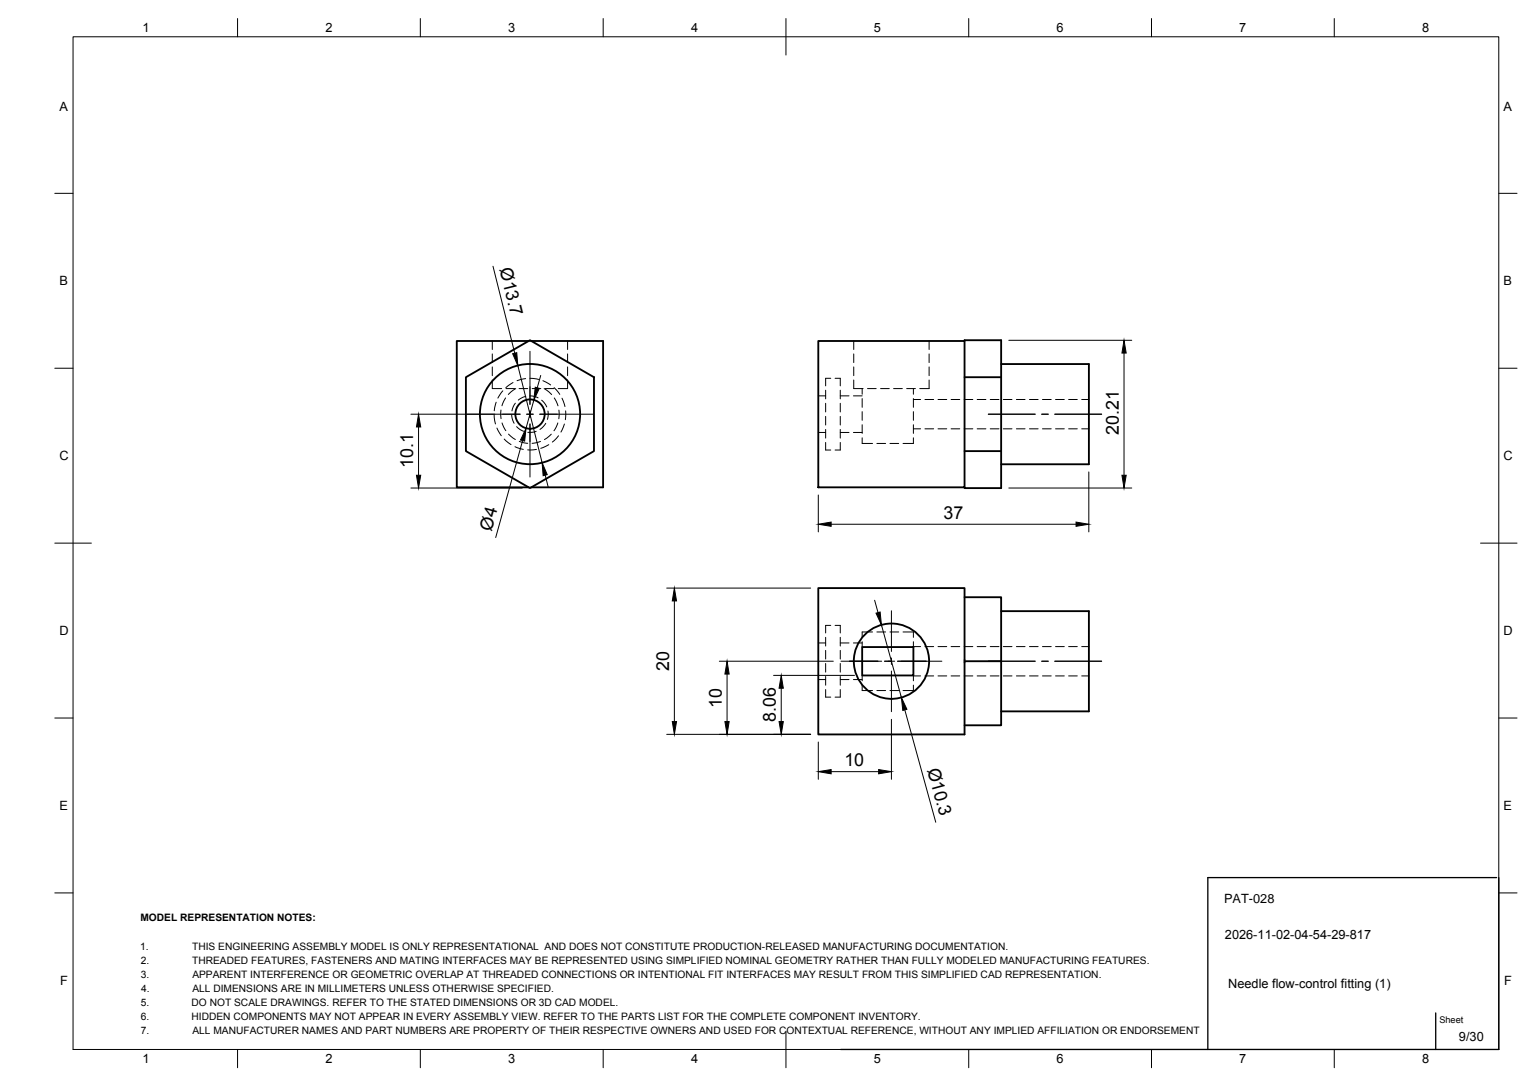
ISO-10303-21;
HEADER;
/* Generated by software containing ST-Developer
 * from STEP Tools, Inc. (www.steptools.com) 
 */

FILE_DESCRIPTION(
/* description */ ('Cylinder foot and clevis mount kit'),
/* implementation_level */ '2;1');

FILE_NAME(
/* name */ 'Needle flow-control fitting (1).step',
/* time_stamp */ '2026-10-27T20:10:43-07:00',
/* author */ (''),
/* organization */ (''),
/* preprocessor_version */ 'ST-DEVELOPER v20.2',
/* originating_system */ 'Autodesk Translation Framework v15.17.0.0',
/* authorisation */ '');

FILE_SCHEMA (('AUTOMOTIVE_DESIGN { 1 0 10303 214 3 1 1 }'));
ENDSEC;

DATA;
#10=MECHANICAL_DESIGN_GEOMETRIC_PRESENTATION_REPRESENTATION('',(#342),#9102);
#286=SHAPE_REPRESENTATION_RELATIONSHIP('SRR','None',#9233,#314);
#314=ADVANCED_BREP_SHAPE_REPRESENTATION('',(#370),#9076);
#342=STYLED_ITEM('',(#9453),#370);
#370=MANIFOLD_SOLID_BREP('Body1',#4928);
#430=FACE_BOUND('',#1139,.T.);
#431=FACE_BOUND('',#1141,.T.);
#432=FACE_BOUND('',#1145,.T.);
#433=FACE_BOUND('',#1147,.T.);
#434=FACE_BOUND('',#1151,.T.);
#435=FACE_BOUND('',#1155,.T.);
#436=FACE_BOUND('',#1159,.T.);
#437=FACE_BOUND('',#1163,.T.);
#438=FACE_BOUND('',#1174,.T.);
#567=PLANE('',#5462);
#568=PLANE('',#5463);
#569=PLANE('',#5471);
#570=PLANE('',#5473);
#571=PLANE('',#5478);
#572=PLANE('',#5480);
#573=PLANE('',#5481);
#574=PLANE('',#5482);
#575=PLANE('',#5483);
#576=PLANE('',#5484);
#577=PLANE('',#5485);
#578=PLANE('',#5486);
#579=PLANE('',#5487);
#580=PLANE('',#5488);
#581=PLANE('',#5490);
#582=PLANE('',#5491);
#583=PLANE('',#5492);
#584=PLANE('',#5493);
#585=PLANE('',#5494);
#586=PLANE('',#5495);
#587=PLANE('',#5496);
#588=PLANE('',#5501);
#793=FACE_OUTER_BOUND('',#1137,.T.);
#794=FACE_OUTER_BOUND('',#1138,.T.);
#795=FACE_OUTER_BOUND('',#1140,.T.);
#796=FACE_OUTER_BOUND('',#1142,.T.);
#797=FACE_OUTER_BOUND('',#1143,.T.);
#798=FACE_OUTER_BOUND('',#1144,.T.);
#799=FACE_OUTER_BOUND('',#1146,.T.);
#800=FACE_OUTER_BOUND('',#1148,.T.);
#801=FACE_OUTER_BOUND('',#1149,.T.);
#802=FACE_OUTER_BOUND('',#1150,.T.);
#803=FACE_OUTER_BOUND('',#1152,.T.);
#804=FACE_OUTER_BOUND('',#1153,.T.);
#805=FACE_OUTER_BOUND('',#1154,.T.);
#806=FACE_OUTER_BOUND('',#1156,.T.);
#807=FACE_OUTER_BOUND('',#1157,.T.);
#808=FACE_OUTER_BOUND('',#1158,.T.);
#809=FACE_OUTER_BOUND('',#1160,.T.);
#810=FACE_OUTER_BOUND('',#1161,.T.);
#811=FACE_OUTER_BOUND('',#1162,.T.);
#812=FACE_OUTER_BOUND('',#1164,.T.);
#813=FACE_OUTER_BOUND('',#1165,.T.);
#814=FACE_OUTER_BOUND('',#1166,.T.);
#815=FACE_OUTER_BOUND('',#1167,.T.);
#816=FACE_OUTER_BOUND('',#1168,.T.);
#817=FACE_OUTER_BOUND('',#1169,.T.);
#818=FACE_OUTER_BOUND('',#1170,.T.);
#819=FACE_OUTER_BOUND('',#1171,.T.);
#820=FACE_OUTER_BOUND('',#1172,.T.);
#821=FACE_OUTER_BOUND('',#1173,.T.);
#1137=EDGE_LOOP('',(#3719,#3720,#3721,#3722));
#1138=EDGE_LOOP('',(#3723));
#1139=EDGE_LOOP('',(#3724,#3725,#3726,#3727));
#1140=EDGE_LOOP('',(#3728,#3729));
#1141=EDGE_LOOP('',(#3730));
#1142=EDGE_LOOP('',(#3731,#3732,#3733,#3734));
#1143=EDGE_LOOP('',(#3735,#3736,#3737,#3738));
#1144=EDGE_LOOP('',(#3739));
#1145=EDGE_LOOP('',(#3740));
#1146=EDGE_LOOP('',(#3741));
#1147=EDGE_LOOP('',(#3742));
#1148=EDGE_LOOP('',(#3743,#3744,#3745,#3746));
#1149=EDGE_LOOP('',(#3747,#3748,#3749,#3750));
#1150=EDGE_LOOP('',(#3751,#3752));
#1151=EDGE_LOOP('',(#3753));
#1152=EDGE_LOOP('',(#3754,#3755,#3756,#3757,#3758,#3759));
#1153=EDGE_LOOP('',(#3760,#3761,#3762,#3763));
#1154=EDGE_LOOP('',(#3764,#3765,#3766,#3767,#3768,#3769));
#1155=EDGE_LOOP('',(#3770));
#1156=EDGE_LOOP('',(#3771,#3772,#3773,#3774));
#1157=EDGE_LOOP('',(#3775,#3776,#3777,#3778,#3779,#3780));
#1158=EDGE_LOOP('',(#3781,#3782,#3783,#3784));
#1159=EDGE_LOOP('',(#3785));
#1160=EDGE_LOOP('',(#3786,#3787,#3788,#3789,#3790,#3791));
#1161=EDGE_LOOP('',(#3792,#3793,#3794));
#1162=EDGE_LOOP('',(#3795,#3796,#3797,#3798,#3799,#3800));
#1163=EDGE_LOOP('',(#3801));
#1164=EDGE_LOOP('',(#3802,#3803,#3804,#3805));
#1165=EDGE_LOOP('',(#3806,#3807,#3808,#3809,#3810));
#1166=EDGE_LOOP('',(#3811,#3812,#3813,#3814,#3815));
#1167=EDGE_LOOP('',(#3816,#3817,#3818,#3819));
#1168=EDGE_LOOP('',(#3820,#3821,#3822,#3823,#3824));
#1169=EDGE_LOOP('',(#3825,#3826,#3827,#3828,#3829));
#1170=EDGE_LOOP('',(#3830,#3831,#3832));
#1171=EDGE_LOOP('',(#3833,#3834,#3835,#3836));
#1172=EDGE_LOOP('',(#3837,#3838,#3839,#3840));
#1173=EDGE_LOOP('',(#3841));
#1174=EDGE_LOOP('',(#3842));
#1521=LINE('',#7931,#1870);
#1522=LINE('',#7936,#1871);
#1523=LINE('',#7938,#1872);
#1524=LINE('',#7940,#1873);
#1525=LINE('',#7941,#1874);
#1526=LINE('',#7952,#1875);
#1527=LINE('',#7961,#1876);
#1528=LINE('',#7964,#1877);
#1529=LINE('',#7972,#1878);
#1530=LINE('',#7974,#1879);
#1531=LINE('',#7976,#1880);
#1532=LINE('',#7978,#1881);
#1533=LINE('',#7980,#1882);
#1534=LINE('',#7981,#1883);
#1535=LINE('',#7985,#1884);
#1536=LINE('',#7987,#1885);
#1537=LINE('',#7989,#1886);
#1538=LINE('',#7990,#1887);
#1539=LINE('',#7993,#1888);
#1540=LINE('',#7994,#1889);
#1541=LINE('',#7996,#1890);
#1542=LINE('',#7997,#1891);
#1543=LINE('',#8000,#1892);
#1544=LINE('',#8001,#1893);
#1545=LINE('',#8004,#1894);
#1546=LINE('',#8005,#1895);
#1547=LINE('',#8006,#1896);
#1548=LINE('',#8010,#1897);
#1549=LINE('',#8012,#1898);
#1550=LINE('',#8013,#1899);
#1551=LINE('',#8016,#1900);
#1552=LINE('',#8017,#1901);
#1553=LINE('',#8021,#1902);
#1554=LINE('',#8023,#1903);
#1555=LINE('',#8025,#1904);
#1556=LINE('',#8027,#1905);
#1557=LINE('',#8029,#1906);
#1558=LINE('',#8030,#1907);
#1559=LINE('',#8034,#1908);
#1560=LINE('',#8035,#1909);
#1561=LINE('',#8038,#1910);
#1562=LINE('',#8039,#1911);
#1563=LINE('',#8041,#1912);
#1564=LINE('',#8042,#1913);
#1565=LINE('',#8044,#1914);
#1566=LINE('',#8046,#1915);
#1567=LINE('',#8051,#1916);
#1568=LINE('',#8055,#1917);
#1870=VECTOR('',#6398,0.515);
#1871=VECTOR('',#6403,1.);
#1872=VECTOR('',#6404,1.);
#1873=VECTOR('',#6405,1.);
#1874=VECTOR('',#6406,1.);
#1875=VECTOR('',#6421,0.49);
#1876=VECTOR('',#6434,0.25);
#1877=VECTOR('',#6437,0.25);
#1878=VECTOR('',#6446,1.);
#1879=VECTOR('',#6447,1.);
#1880=VECTOR('',#6448,1.);
#1881=VECTOR('',#6449,1.);
#1882=VECTOR('',#6450,1.);
#1883=VECTOR('',#6451,1.);
#1884=VECTOR('',#6454,1.);
#1885=VECTOR('',#6455,1.);
#1886=VECTOR('',#6456,1.);
#1887=VECTOR('',#6457,1.);
#1888=VECTOR('',#6460,1.);
#1889=VECTOR('',#6461,1.);
#1890=VECTOR('',#6462,1.);
#1891=VECTOR('',#6463,1.);
#1892=VECTOR('',#6466,1.);
#1893=VECTOR('',#6467,1.);
#1894=VECTOR('',#6470,1.);
#1895=VECTOR('',#6471,1.);
#1896=VECTOR('',#6472,1.);
#1897=VECTOR('',#6477,1.);
#1898=VECTOR('',#6478,1.);
#1899=VECTOR('',#6479,1.);
#1900=VECTOR('',#6482,1.);
#1901=VECTOR('',#6483,1.);
#1902=VECTOR('',#6486,1.);
#1903=VECTOR('',#6487,1.);
#1904=VECTOR('',#6488,1.);
#1905=VECTOR('',#6489,1.);
#1906=VECTOR('',#6490,1.);
#1907=VECTOR('',#6491,1.);
#1908=VECTOR('',#6496,1.);
#1909=VECTOR('',#6497,1.);
#1910=VECTOR('',#6500,1.);
#1911=VECTOR('',#6501,1.);
#1912=VECTOR('',#6504,1.);
#1913=VECTOR('',#6505,1.);
#1914=VECTOR('',#6508,1.);
#1915=VECTOR('',#6511,1.);
#1916=VECTOR('',#6518,0.2);
#1917=VECTOR('',#6523,0.685);
#2185=CIRCLE('',#5460,0.515);
#2186=CIRCLE('',#5461,0.515);
#2187=CIRCLE('',#5464,0.4);
#2188=CIRCLE('',#5465,0.25);
#2189=CIRCLE('',#5467,0.4);
#2190=CIRCLE('',#5469,0.49);
#2191=CIRCLE('',#5470,0.49);
#2192=CIRCLE('',#5472,0.25);
#2193=CIRCLE('',#5474,0.25);
#2194=CIRCLE('',#5477,0.25);
#2195=CIRCLE('',#5479,0.2);
#2196=CIRCLE('',#5489,0.685);
#2197=CIRCLE('',#5498,0.2);
#2198=CIRCLE('',#5500,0.685);
#2452=VERTEX_POINT('',#7928);
#2453=VERTEX_POINT('',#7930);
#2454=VERTEX_POINT('',#7934);
#2455=VERTEX_POINT('',#7935);
#2456=VERTEX_POINT('',#7937);
#2457=VERTEX_POINT('',#7939);
#2458=VERTEX_POINT('',#7944);
#2459=VERTEX_POINT('',#7949);
#2460=VERTEX_POINT('',#7951);
#2461=VERTEX_POINT('',#7955);
#2462=VERTEX_POINT('',#7958);
#2463=VERTEX_POINT('',#7963);
#2464=VERTEX_POINT('',#7967);
#2465=VERTEX_POINT('',#7970);
#2466=VERTEX_POINT('',#7971);
#2467=VERTEX_POINT('',#7973);
#2468=VERTEX_POINT('',#7975);
#2469=VERTEX_POINT('',#7977);
#2470=VERTEX_POINT('',#7979);
#2471=VERTEX_POINT('',#7983);
#2472=VERTEX_POINT('',#7984);
#2473=VERTEX_POINT('',#7986);
#2474=VERTEX_POINT('',#7988);
#2475=VERTEX_POINT('',#7992);
#2476=VERTEX_POINT('',#7995);
#2477=VERTEX_POINT('',#7999);
#2478=VERTEX_POINT('',#8003);
#2479=VERTEX_POINT('',#8009);
#2480=VERTEX_POINT('',#8011);
#2481=VERTEX_POINT('',#8015);
#2482=VERTEX_POINT('',#8019);
#2483=VERTEX_POINT('',#8020);
#2484=VERTEX_POINT('',#8022);
#2485=VERTEX_POINT('',#8024);
#2486=VERTEX_POINT('',#8026);
#2487=VERTEX_POINT('',#8028);
#2488=VERTEX_POINT('',#8031);
#2489=VERTEX_POINT('',#8037);
#2490=VERTEX_POINT('',#8050);
#2491=VERTEX_POINT('',#8054);
#2914=EDGE_CURVE('',#2452,#2452,#2185,.T.);
#2915=EDGE_CURVE('',#2452,#2453,#1521,.T.);
#2916=EDGE_CURVE('',#2453,#2453,#2186,.T.);
#2917=EDGE_CURVE('',#2454,#2455,#1522,.T.);
#2918=EDGE_CURVE('',#2456,#2454,#1523,.T.);
#2919=EDGE_CURVE('',#2457,#2456,#1524,.T.);
#2920=EDGE_CURVE('',#2455,#2457,#1525,.T.);
#2921=EDGE_CURVE('',#2456,#2454,#2187,.T.);
#2922=EDGE_CURVE('',#2458,#2458,#2188,.T.);
#2923=EDGE_CURVE('',#2457,#2455,#2189,.T.);
#2924=EDGE_CURVE('',#2459,#2459,#2190,.T.);
#2925=EDGE_CURVE('',#2459,#2460,#1526,.T.);
#2926=EDGE_CURVE('',#2460,#2460,#2191,.T.);
#2927=EDGE_CURVE('',#2461,#2461,#2192,.T.);
#2928=EDGE_CURVE('',#2462,#2462,#2193,.T.);
#2929=EDGE_CURVE('',#2458,#2462,#1527,.T.);
#2930=EDGE_CURVE('',#2461,#2463,#1528,.T.);
#2931=EDGE_CURVE('',#2463,#2463,#2194,.T.);
#2932=EDGE_CURVE('',#2464,#2464,#2195,.T.);
#2933=EDGE_CURVE('',#2465,#2466,#1529,.T.);
#2934=EDGE_CURVE('',#2466,#2467,#1530,.T.);
#2935=EDGE_CURVE('',#2467,#2468,#1531,.T.);
#2936=EDGE_CURVE('',#2469,#2468,#1532,.T.);
#2937=EDGE_CURVE('',#2470,#2469,#1533,.T.);
#2938=EDGE_CURVE('',#2465,#2470,#1534,.T.);
#2939=EDGE_CURVE('',#2471,#2472,#1535,.T.);
#2940=EDGE_CURVE('',#2472,#2473,#1536,.T.);
#2941=EDGE_CURVE('',#2474,#2473,#1537,.T.);
#2942=EDGE_CURVE('',#2471,#2474,#1538,.T.);
#2943=EDGE_CURVE('',#2475,#2468,#1539,.T.);
#2944=EDGE_CURVE('',#2475,#2471,#1540,.T.);
#2945=EDGE_CURVE('',#2476,#2474,#1541,.T.);
#2946=EDGE_CURVE('',#2469,#2476,#1542,.T.);
#2947=EDGE_CURVE('',#2477,#2476,#1543,.T.);
#2948=EDGE_CURVE('',#2470,#2477,#1544,.T.);
#2949=EDGE_CURVE('',#2472,#2478,#1545,.T.);
#2950=EDGE_CURVE('',#2465,#2478,#1546,.T.);
#2951=EDGE_CURVE('',#2473,#2477,#1547,.T.);
#2952=EDGE_CURVE('',#2479,#2478,#1548,.T.);
#2953=EDGE_CURVE('',#2475,#2480,#1549,.T.);
#2954=EDGE_CURVE('',#2480,#2479,#1550,.T.);
#2955=EDGE_CURVE('',#2468,#2481,#1551,.T.);
#2956=EDGE_CURVE('',#2481,#2475,#1552,.T.);
#2957=EDGE_CURVE('',#2482,#2483,#1553,.T.);
#2958=EDGE_CURVE('',#2484,#2482,#1554,.T.);
#2959=EDGE_CURVE('',#2485,#2484,#1555,.T.);
#2960=EDGE_CURVE('',#2486,#2485,#1556,.T.);
#2961=EDGE_CURVE('',#2487,#2486,#1557,.T.);
#2962=EDGE_CURVE('',#2483,#2487,#1558,.T.);
#2963=EDGE_CURVE('',#2488,#2488,#2196,.T.);
#2964=EDGE_CURVE('',#2482,#2467,#1559,.T.);
#2965=EDGE_CURVE('',#2484,#2466,#1560,.T.);
#2966=EDGE_CURVE('',#2489,#2465,#1561,.T.);
#2967=EDGE_CURVE('',#2485,#2489,#1562,.T.);
#2968=EDGE_CURVE('',#2478,#2489,#1563,.T.);
#2969=EDGE_CURVE('',#2486,#2479,#1564,.T.);
#2970=EDGE_CURVE('',#2487,#2480,#1565,.T.);
#2971=EDGE_CURVE('',#2483,#2481,#1566,.T.);
#2972=EDGE_CURVE('',#2464,#2490,#1567,.T.);
#2973=EDGE_CURVE('',#2490,#2490,#2197,.T.);
#2974=EDGE_CURVE('',#2488,#2491,#1568,.T.);
#2975=EDGE_CURVE('',#2491,#2491,#2198,.T.);
#3719=ORIENTED_EDGE('',*,*,#2914,.F.);
#3720=ORIENTED_EDGE('',*,*,#2915,.T.);
#3721=ORIENTED_EDGE('',*,*,#2916,.F.);
#3722=ORIENTED_EDGE('',*,*,#2915,.F.);
#3723=ORIENTED_EDGE('',*,*,#2914,.T.);
#3724=ORIENTED_EDGE('',*,*,#2917,.F.);
#3725=ORIENTED_EDGE('',*,*,#2918,.F.);
#3726=ORIENTED_EDGE('',*,*,#2919,.F.);
#3727=ORIENTED_EDGE('',*,*,#2920,.F.);
#3728=ORIENTED_EDGE('',*,*,#2918,.T.);
#3729=ORIENTED_EDGE('',*,*,#2921,.F.);
#3730=ORIENTED_EDGE('',*,*,#2922,.T.);
#3731=ORIENTED_EDGE('',*,*,#2919,.T.);
#3732=ORIENTED_EDGE('',*,*,#2921,.T.);
#3733=ORIENTED_EDGE('',*,*,#2917,.T.);
#3734=ORIENTED_EDGE('',*,*,#2923,.F.);
#3735=ORIENTED_EDGE('',*,*,#2924,.F.);
#3736=ORIENTED_EDGE('',*,*,#2925,.T.);
#3737=ORIENTED_EDGE('',*,*,#2926,.T.);
#3738=ORIENTED_EDGE('',*,*,#2925,.F.);
#3739=ORIENTED_EDGE('',*,*,#2926,.F.);
#3740=ORIENTED_EDGE('',*,*,#2927,.F.);
#3741=ORIENTED_EDGE('',*,*,#2924,.T.);
#3742=ORIENTED_EDGE('',*,*,#2928,.F.);
#3743=ORIENTED_EDGE('',*,*,#2922,.F.);
#3744=ORIENTED_EDGE('',*,*,#2929,.T.);
#3745=ORIENTED_EDGE('',*,*,#2928,.T.);
#3746=ORIENTED_EDGE('',*,*,#2929,.F.);
#3747=ORIENTED_EDGE('',*,*,#2927,.T.);
#3748=ORIENTED_EDGE('',*,*,#2930,.T.);
#3749=ORIENTED_EDGE('',*,*,#2931,.F.);
#3750=ORIENTED_EDGE('',*,*,#2930,.F.);
#3751=ORIENTED_EDGE('',*,*,#2920,.T.);
#3752=ORIENTED_EDGE('',*,*,#2923,.T.);
#3753=ORIENTED_EDGE('',*,*,#2932,.F.);
#3754=ORIENTED_EDGE('',*,*,#2933,.T.);
#3755=ORIENTED_EDGE('',*,*,#2934,.T.);
#3756=ORIENTED_EDGE('',*,*,#2935,.T.);
#3757=ORIENTED_EDGE('',*,*,#2936,.F.);
#3758=ORIENTED_EDGE('',*,*,#2937,.F.);
#3759=ORIENTED_EDGE('',*,*,#2938,.F.);
#3760=ORIENTED_EDGE('',*,*,#2939,.T.);
#3761=ORIENTED_EDGE('',*,*,#2940,.T.);
#3762=ORIENTED_EDGE('',*,*,#2941,.F.);
#3763=ORIENTED_EDGE('',*,*,#2942,.F.);
#3764=ORIENTED_EDGE('',*,*,#2936,.T.);
#3765=ORIENTED_EDGE('',*,*,#2943,.F.);
#3766=ORIENTED_EDGE('',*,*,#2944,.T.);
#3767=ORIENTED_EDGE('',*,*,#2942,.T.);
#3768=ORIENTED_EDGE('',*,*,#2945,.F.);
#3769=ORIENTED_EDGE('',*,*,#2946,.F.);
#3770=ORIENTED_EDGE('',*,*,#2916,.T.);
#3771=ORIENTED_EDGE('',*,*,#2937,.T.);
#3772=ORIENTED_EDGE('',*,*,#2946,.T.);
#3773=ORIENTED_EDGE('',*,*,#2947,.F.);
#3774=ORIENTED_EDGE('',*,*,#2948,.F.);
#3775=ORIENTED_EDGE('',*,*,#2949,.T.);
#3776=ORIENTED_EDGE('',*,*,#2950,.F.);
#3777=ORIENTED_EDGE('',*,*,#2938,.T.);
#3778=ORIENTED_EDGE('',*,*,#2948,.T.);
#3779=ORIENTED_EDGE('',*,*,#2951,.F.);
#3780=ORIENTED_EDGE('',*,*,#2940,.F.);
#3781=ORIENTED_EDGE('',*,*,#2951,.T.);
#3782=ORIENTED_EDGE('',*,*,#2947,.T.);
#3783=ORIENTED_EDGE('',*,*,#2945,.T.);
#3784=ORIENTED_EDGE('',*,*,#2941,.T.);
#3785=ORIENTED_EDGE('',*,*,#2931,.T.);
#3786=ORIENTED_EDGE('',*,*,#2952,.T.);
#3787=ORIENTED_EDGE('',*,*,#2949,.F.);
#3788=ORIENTED_EDGE('',*,*,#2939,.F.);
#3789=ORIENTED_EDGE('',*,*,#2944,.F.);
#3790=ORIENTED_EDGE('',*,*,#2953,.T.);
#3791=ORIENTED_EDGE('',*,*,#2954,.T.);
#3792=ORIENTED_EDGE('',*,*,#2943,.T.);
#3793=ORIENTED_EDGE('',*,*,#2955,.T.);
#3794=ORIENTED_EDGE('',*,*,#2956,.T.);
#3795=ORIENTED_EDGE('',*,*,#2957,.F.);
#3796=ORIENTED_EDGE('',*,*,#2958,.F.);
#3797=ORIENTED_EDGE('',*,*,#2959,.F.);
#3798=ORIENTED_EDGE('',*,*,#2960,.F.);
#3799=ORIENTED_EDGE('',*,*,#2961,.F.);
#3800=ORIENTED_EDGE('',*,*,#2962,.F.);
#3801=ORIENTED_EDGE('',*,*,#2963,.T.);
#3802=ORIENTED_EDGE('',*,*,#2958,.T.);
#3803=ORIENTED_EDGE('',*,*,#2964,.T.);
#3804=ORIENTED_EDGE('',*,*,#2934,.F.);
#3805=ORIENTED_EDGE('',*,*,#2965,.F.);
#3806=ORIENTED_EDGE('',*,*,#2959,.T.);
#3807=ORIENTED_EDGE('',*,*,#2965,.T.);
#3808=ORIENTED_EDGE('',*,*,#2933,.F.);
#3809=ORIENTED_EDGE('',*,*,#2966,.F.);
#3810=ORIENTED_EDGE('',*,*,#2967,.F.);
#3811=ORIENTED_EDGE('',*,*,#2960,.T.);
#3812=ORIENTED_EDGE('',*,*,#2967,.T.);
#3813=ORIENTED_EDGE('',*,*,#2968,.F.);
#3814=ORIENTED_EDGE('',*,*,#2952,.F.);
#3815=ORIENTED_EDGE('',*,*,#2969,.F.);
#3816=ORIENTED_EDGE('',*,*,#2961,.T.);
#3817=ORIENTED_EDGE('',*,*,#2969,.T.);
#3818=ORIENTED_EDGE('',*,*,#2954,.F.);
#3819=ORIENTED_EDGE('',*,*,#2970,.F.);
#3820=ORIENTED_EDGE('',*,*,#2962,.T.);
#3821=ORIENTED_EDGE('',*,*,#2970,.T.);
#3822=ORIENTED_EDGE('',*,*,#2953,.F.);
#3823=ORIENTED_EDGE('',*,*,#2956,.F.);
#3824=ORIENTED_EDGE('',*,*,#2971,.F.);
#3825=ORIENTED_EDGE('',*,*,#2957,.T.);
#3826=ORIENTED_EDGE('',*,*,#2971,.T.);
#3827=ORIENTED_EDGE('',*,*,#2955,.F.);
#3828=ORIENTED_EDGE('',*,*,#2935,.F.);
#3829=ORIENTED_EDGE('',*,*,#2964,.F.);
#3830=ORIENTED_EDGE('',*,*,#2950,.T.);
#3831=ORIENTED_EDGE('',*,*,#2968,.T.);
#3832=ORIENTED_EDGE('',*,*,#2966,.T.);
#3833=ORIENTED_EDGE('',*,*,#2932,.T.);
#3834=ORIENTED_EDGE('',*,*,#2972,.T.);
#3835=ORIENTED_EDGE('',*,*,#2973,.T.);
#3836=ORIENTED_EDGE('',*,*,#2972,.F.);
#3837=ORIENTED_EDGE('',*,*,#2963,.F.);
#3838=ORIENTED_EDGE('',*,*,#2974,.T.);
#3839=ORIENTED_EDGE('',*,*,#2975,.T.);
#3840=ORIENTED_EDGE('',*,*,#2974,.F.);
#3841=ORIENTED_EDGE('',*,*,#2975,.F.);
#3842=ORIENTED_EDGE('',*,*,#2973,.F.);
#4559=CYLINDRICAL_SURFACE('',#5459,0.515);
#4560=CYLINDRICAL_SURFACE('',#5466,0.4);
#4561=CYLINDRICAL_SURFACE('',#5468,0.49);
#4562=CYLINDRICAL_SURFACE('',#5475,0.25);
#4563=CYLINDRICAL_SURFACE('',#5476,0.25);
#4564=CYLINDRICAL_SURFACE('',#5497,0.2);
#4565=CYLINDRICAL_SURFACE('',#5499,0.685);
#4716=ADVANCED_FACE('',(#793),#4559,.F.);
#4717=ADVANCED_FACE('',(#794,#430),#567,.T.);
#4718=ADVANCED_FACE('',(#795,#431),#568,.F.);
#4719=ADVANCED_FACE('',(#796),#4560,.F.);
#4720=ADVANCED_FACE('',(#797),#4561,.F.);
#4721=ADVANCED_FACE('',(#798,#432),#569,.F.);
#4722=ADVANCED_FACE('',(#799,#433),#570,.T.);
#4723=ADVANCED_FACE('',(#800),#4562,.F.);
#4724=ADVANCED_FACE('',(#801),#4563,.F.);
#4725=ADVANCED_FACE('',(#802,#434),#571,.T.);
#4726=ADVANCED_FACE('',(#803),#572,.F.);
#4727=ADVANCED_FACE('',(#804),#573,.T.);
#4728=ADVANCED_FACE('',(#805,#435),#574,.T.);
#4729=ADVANCED_FACE('',(#806),#575,.T.);
#4730=ADVANCED_FACE('',(#807),#576,.T.);
#4731=ADVANCED_FACE('',(#808,#436),#577,.T.);
#4732=ADVANCED_FACE('',(#809),#578,.F.);
#4733=ADVANCED_FACE('',(#810),#579,.T.);
#4734=ADVANCED_FACE('',(#811,#437),#580,.F.);
#4735=ADVANCED_FACE('',(#812),#581,.T.);
#4736=ADVANCED_FACE('',(#813),#582,.T.);
#4737=ADVANCED_FACE('',(#814),#583,.T.);
#4738=ADVANCED_FACE('',(#815),#584,.T.);
#4739=ADVANCED_FACE('',(#816),#585,.T.);
#4740=ADVANCED_FACE('',(#817),#586,.T.);
#4741=ADVANCED_FACE('',(#818),#587,.T.);
#4742=ADVANCED_FACE('',(#819),#4564,.F.);
#4743=ADVANCED_FACE('',(#820),#4565,.T.);
#4744=ADVANCED_FACE('',(#821,#438),#588,.F.);
#4928=CLOSED_SHELL('',(#4716,#4717,#4718,#4719,#4720,#4721,#4722,#4723,
#4724,#4725,#4726,#4727,#4728,#4729,#4730,#4731,#4732,#4733,#4734,#4735,
#4736,#4737,#4738,#4739,#4740,#4741,#4742,#4743,#4744));
#5458=AXIS2_PLACEMENT_3D('',#7926,#6392,#6393);
#5459=AXIS2_PLACEMENT_3D('',#7927,#6394,#6395);
#5460=AXIS2_PLACEMENT_3D('',#7929,#6396,#6397);
#5461=AXIS2_PLACEMENT_3D('',#7932,#6399,#6400);
#5462=AXIS2_PLACEMENT_3D('',#7933,#6401,#6402);
#5463=AXIS2_PLACEMENT_3D('',#7942,#6407,#6408);
#5464=AXIS2_PLACEMENT_3D('',#7943,#6409,#6410);
#5465=AXIS2_PLACEMENT_3D('',#7945,#6411,#6412);
#5466=AXIS2_PLACEMENT_3D('',#7946,#6413,#6414);
#5467=AXIS2_PLACEMENT_3D('',#7947,#6415,#6416);
#5468=AXIS2_PLACEMENT_3D('',#7948,#6417,#6418);
#5469=AXIS2_PLACEMENT_3D('',#7950,#6419,#6420);
#5470=AXIS2_PLACEMENT_3D('',#7953,#6422,#6423);
#5471=AXIS2_PLACEMENT_3D('',#7954,#6424,#6425);
#5472=AXIS2_PLACEMENT_3D('',#7956,#6426,#6427);
#5473=AXIS2_PLACEMENT_3D('',#7957,#6428,#6429);
#5474=AXIS2_PLACEMENT_3D('',#7959,#6430,#6431);
#5475=AXIS2_PLACEMENT_3D('',#7960,#6432,#6433);
#5476=AXIS2_PLACEMENT_3D('',#7962,#6435,#6436);
#5477=AXIS2_PLACEMENT_3D('',#7965,#6438,#6439);
#5478=AXIS2_PLACEMENT_3D('',#7966,#6440,#6441);
#5479=AXIS2_PLACEMENT_3D('',#7968,#6442,#6443);
#5480=AXIS2_PLACEMENT_3D('',#7969,#6444,#6445);
#5481=AXIS2_PLACEMENT_3D('',#7982,#6452,#6453);
#5482=AXIS2_PLACEMENT_3D('',#7991,#6458,#6459);
#5483=AXIS2_PLACEMENT_3D('',#7998,#6464,#6465);
#5484=AXIS2_PLACEMENT_3D('',#8002,#6468,#6469);
#5485=AXIS2_PLACEMENT_3D('',#8007,#6473,#6474);
#5486=AXIS2_PLACEMENT_3D('',#8008,#6475,#6476);
#5487=AXIS2_PLACEMENT_3D('',#8014,#6480,#6481);
#5488=AXIS2_PLACEMENT_3D('',#8018,#6484,#6485);
#5489=AXIS2_PLACEMENT_3D('',#8032,#6492,#6493);
#5490=AXIS2_PLACEMENT_3D('',#8033,#6494,#6495);
#5491=AXIS2_PLACEMENT_3D('',#8036,#6498,#6499);
#5492=AXIS2_PLACEMENT_3D('',#8040,#6502,#6503);
#5493=AXIS2_PLACEMENT_3D('',#8043,#6506,#6507);
#5494=AXIS2_PLACEMENT_3D('',#8045,#6509,#6510);
#5495=AXIS2_PLACEMENT_3D('',#8047,#6512,#6513);
#5496=AXIS2_PLACEMENT_3D('',#8048,#6514,#6515);
#5497=AXIS2_PLACEMENT_3D('',#8049,#6516,#6517);
#5498=AXIS2_PLACEMENT_3D('',#8052,#6519,#6520);
#5499=AXIS2_PLACEMENT_3D('',#8053,#6521,#6522);
#5500=AXIS2_PLACEMENT_3D('',#8056,#6524,#6525);
#5501=AXIS2_PLACEMENT_3D('',#8057,#6526,#6527);
#6392=DIRECTION('axis',(0.,0.,1.));
#6393=DIRECTION('refdir',(1.,0.,0.));
#6394=DIRECTION('center_axis',(1.,0.,0.));
#6395=DIRECTION('ref_axis',(0.,0.,-1.));
#6396=DIRECTION('center_axis',(1.,0.,0.));
#6397=DIRECTION('ref_axis',(0.,0.,-1.));
#6398=DIRECTION('',(1.,0.,0.));
#6399=DIRECTION('center_axis',(-1.,0.,0.));
#6400=DIRECTION('ref_axis',(0.,0.,-1.));
#6401=DIRECTION('center_axis',(1.,0.,0.));
#6402=DIRECTION('ref_axis',(0.,0.,-1.));
#6403=DIRECTION('',(0.,0.,-1.));
#6404=DIRECTION('',(0.,-1.,0.));
#6405=DIRECTION('',(0.,0.,1.));
#6406=DIRECTION('',(0.,1.,0.));
#6407=DIRECTION('center_axis',(0.,0.,1.));
#6408=DIRECTION('ref_axis',(1.,0.,0.));
#6409=DIRECTION('center_axis',(0.,0.,1.));
#6410=DIRECTION('ref_axis',(1.,0.,0.));
#6411=DIRECTION('center_axis',(0.,0.,1.));
#6412=DIRECTION('ref_axis',(1.,0.,0.));
#6413=DIRECTION('center_axis',(0.,0.,1.));
#6414=DIRECTION('ref_axis',(-1.,1.22464679914735E-16,0.));
#6415=DIRECTION('center_axis',(0.,0.,1.));
#6416=DIRECTION('ref_axis',(1.,0.,0.));
#6417=DIRECTION('center_axis',(0.,0.,1.));
#6418=DIRECTION('ref_axis',(1.,0.,0.));
#6419=DIRECTION('center_axis',(0.,0.,1.));
#6420=DIRECTION('ref_axis',(1.,0.,0.));
#6421=DIRECTION('',(0.,0.,1.));
#6422=DIRECTION('center_axis',(0.,0.,1.));
#6423=DIRECTION('ref_axis',(1.,0.,0.));
#6424=DIRECTION('center_axis',(0.,0.,1.));
#6425=DIRECTION('ref_axis',(1.,0.,0.));
#6426=DIRECTION('center_axis',(0.,0.,-1.));
#6427=DIRECTION('ref_axis',(1.,0.,0.));
#6428=DIRECTION('center_axis',(0.,0.,1.));
#6429=DIRECTION('ref_axis',(1.,0.,0.));
#6430=DIRECTION('center_axis',(0.,0.,1.));
#6431=DIRECTION('ref_axis',(1.,0.,0.));
#6432=DIRECTION('center_axis',(0.,0.,1.));
#6433=DIRECTION('ref_axis',(1.,0.,0.));
#6434=DIRECTION('',(0.,0.,1.));
#6435=DIRECTION('center_axis',(0.,0.,1.));
#6436=DIRECTION('ref_axis',(1.,0.,0.));
#6437=DIRECTION('',(0.,0.,1.));
#6438=DIRECTION('center_axis',(0.,0.,-1.));
#6439=DIRECTION('ref_axis',(1.,0.,0.));
#6440=DIRECTION('center_axis',(0.,0.,1.));
#6441=DIRECTION('ref_axis',(1.,0.,0.));
#6442=DIRECTION('center_axis',(0.,0.,1.));
#6443=DIRECTION('ref_axis',(1.,0.,0.));
#6444=DIRECTION('center_axis',(0.,0.,1.));
#6445=DIRECTION('ref_axis',(1.,0.,0.));
#6446=DIRECTION('',(0.5,-0.866025403784439,0.));
#6447=DIRECTION('',(1.,0.,0.));
#6448=DIRECTION('',(0.5,0.866025403784439,0.));
#6449=DIRECTION('',(0.,1.,0.));
#6450=DIRECTION('',(1.,0.,0.));
#6451=DIRECTION('',(0.,-1.,0.));
#6452=DIRECTION('center_axis',(0.,1.,0.));
#6453=DIRECTION('ref_axis',(-1.,0.,0.));
#6454=DIRECTION('',(-1.,0.,0.));
#6455=DIRECTION('',(0.,0.,1.));
#6456=DIRECTION('',(-1.,0.,0.));
#6457=DIRECTION('',(0.,0.,1.));
#6458=DIRECTION('center_axis',(1.,0.,0.));
#6459=DIRECTION('ref_axis',(0.,1.,0.));
#6460=DIRECTION('',(0.,-1.,0.));
#6461=DIRECTION('',(0.,1.,0.));
#6462=DIRECTION('',(0.,1.,0.));
#6463=DIRECTION('',(0.,0.,1.));
#6464=DIRECTION('center_axis',(0.,-1.,0.));
#6465=DIRECTION('ref_axis',(1.,0.,0.));
#6466=DIRECTION('',(1.,0.,0.));
#6467=DIRECTION('',(0.,0.,1.));
#6468=DIRECTION('center_axis',(-1.,0.,0.));
#6469=DIRECTION('ref_axis',(0.,-1.,0.));
#6470=DIRECTION('',(0.,-1.,0.));
#6471=DIRECTION('',(0.,1.,0.));
#6472=DIRECTION('',(0.,-1.,0.));
#6473=DIRECTION('center_axis',(0.,0.,1.));
#6474=DIRECTION('ref_axis',(1.,0.,0.));
#6475=DIRECTION('center_axis',(0.,0.,1.));
#6476=DIRECTION('ref_axis',(1.,0.,0.));
#6477=DIRECTION('',(-0.5,-0.866025403784439,0.));
#6478=DIRECTION('',(-0.5,0.866025403784439,0.));
#6479=DIRECTION('',(-1.,0.,0.));
#6480=DIRECTION('center_axis',(0.,0.,1.));
#6481=DIRECTION('ref_axis',(1.,0.,0.));
#6482=DIRECTION('',(0.5,0.866025403784439,0.));
#6483=DIRECTION('',(-0.5,0.866025403784439,0.));
#6484=DIRECTION('center_axis',(0.,0.,1.));
#6485=DIRECTION('ref_axis',(1.,0.,0.));
#6486=DIRECTION('',(0.5,0.866025403784439,0.));
#6487=DIRECTION('',(1.,0.,0.));
#6488=DIRECTION('',(0.5,-0.866025403784439,0.));
#6489=DIRECTION('',(-0.5,-0.866025403784439,0.));
#6490=DIRECTION('',(-1.,0.,0.));
#6491=DIRECTION('',(-0.5,0.866025403784439,0.));
#6492=DIRECTION('center_axis',(0.,0.,1.));
#6493=DIRECTION('ref_axis',(1.,0.,0.));
#6494=DIRECTION('center_axis',(0.,-1.,0.));
#6495=DIRECTION('ref_axis',(1.,0.,0.));
#6496=DIRECTION('',(0.,0.,1.));
#6497=DIRECTION('',(0.,0.,1.));
#6498=DIRECTION('center_axis',(-0.866025403784439,-0.5,0.));
#6499=DIRECTION('ref_axis',(0.5,-0.866025403784439,0.));
#6500=DIRECTION('',(0.5,-0.866025403784439,0.));
#6501=DIRECTION('',(0.,0.,1.));
#6502=DIRECTION('center_axis',(-0.866025403784439,0.5,0.));
#6503=DIRECTION('ref_axis',(-0.5,-0.866025403784439,0.));
#6504=DIRECTION('',(-0.5,-0.866025403784439,0.));
#6505=DIRECTION('',(0.,0.,1.));
#6506=DIRECTION('center_axis',(0.,1.,0.));
#6507=DIRECTION('ref_axis',(-1.,0.,0.));
#6508=DIRECTION('',(0.,0.,1.));
#6509=DIRECTION('center_axis',(0.866025403784439,0.5,0.));
#6510=DIRECTION('ref_axis',(-0.5,0.866025403784439,0.));
#6511=DIRECTION('',(0.,0.,1.));
#6512=DIRECTION('center_axis',(0.866025403784439,-0.5,0.));
#6513=DIRECTION('ref_axis',(0.5,0.866025403784439,0.));
#6514=DIRECTION('center_axis',(0.,0.,1.));
#6515=DIRECTION('ref_axis',(1.,0.,0.));
#6516=DIRECTION('center_axis',(0.,0.,1.));
#6517=DIRECTION('ref_axis',(1.,0.,0.));
#6518=DIRECTION('',(0.,0.,-1.));
#6519=DIRECTION('center_axis',(0.,0.,-1.));
#6520=DIRECTION('ref_axis',(1.,0.,0.));
#6521=DIRECTION('center_axis',(0.,0.,1.));
#6522=DIRECTION('ref_axis',(1.,0.,0.));
#6523=DIRECTION('',(0.,0.,-1.));
#6524=DIRECTION('center_axis',(0.,0.,1.));
#6525=DIRECTION('ref_axis',(1.,0.,0.));
#6526=DIRECTION('center_axis',(0.,0.,1.));
#6527=DIRECTION('ref_axis',(1.,0.,0.));
#7926=CARTESIAN_POINT('',(0.,0.,0.));
#7927=CARTESIAN_POINT('Origin',(0.35,11.8,8.5));
#7928=CARTESIAN_POINT('',(0.35,11.8,9.015));
#7929=CARTESIAN_POINT('Origin',(0.35,11.8,8.5));
#7930=CARTESIAN_POINT('',(1.,11.8,9.015));
#7931=CARTESIAN_POINT('',(0.35,11.8,9.015));
#7932=CARTESIAN_POINT('Origin',(1.,11.8,8.5));
#7933=CARTESIAN_POINT('Origin',(0.35,11.8,8.5));
#7934=CARTESIAN_POINT('',(0.35,11.6063508326896,8.9));
#7935=CARTESIAN_POINT('',(0.35,11.6063508326896,8.2));
#7936=CARTESIAN_POINT('',(0.35,11.6063508326896,8.2));
#7937=CARTESIAN_POINT('',(0.35,11.9936491673104,8.9));
#7938=CARTESIAN_POINT('',(0.35,11.8,8.9));
#7939=CARTESIAN_POINT('',(0.35,11.9936491673104,8.2));
#7940=CARTESIAN_POINT('',(0.35,11.9936491673104,8.2));
#7941=CARTESIAN_POINT('',(0.35,11.8,8.2));
#7942=CARTESIAN_POINT('Origin',(0.,11.8,8.9));
#7943=CARTESIAN_POINT('Origin',(0.,11.8,8.9));
#7944=CARTESIAN_POINT('',(-0.25,11.8,8.9));
#7945=CARTESIAN_POINT('Origin',(0.,11.8,8.9));
#7946=CARTESIAN_POINT('Origin',(0.,11.8,8.2));
#7947=CARTESIAN_POINT('Origin',(0.,11.8,8.2));
#7948=CARTESIAN_POINT('Origin',(0.,11.8,9.2));
#7949=CARTESIAN_POINT('',(-0.49,11.8,9.2));
#7950=CARTESIAN_POINT('Origin',(0.,11.8,9.2));
#7951=CARTESIAN_POINT('',(-0.49,11.8,9.4));
#7952=CARTESIAN_POINT('',(-0.49,11.8,9.2));
#7953=CARTESIAN_POINT('Origin',(0.,11.8,9.4));
#7954=CARTESIAN_POINT('Origin',(0.,11.8,9.4));
#7955=CARTESIAN_POINT('',(-0.25,11.8,9.4));
#7956=CARTESIAN_POINT('Origin',(0.,11.8,9.4));
#7957=CARTESIAN_POINT('Origin',(0.,11.8,9.2));
#7958=CARTESIAN_POINT('',(-0.25,11.8,9.2));
#7959=CARTESIAN_POINT('Origin',(0.,11.8,9.2));
#7960=CARTESIAN_POINT('Origin',(0.,11.8,8.8));
#7961=CARTESIAN_POINT('',(-0.25,11.8,8.8));
#7962=CARTESIAN_POINT('Origin',(0.,11.8,8.8));
#7963=CARTESIAN_POINT('',(-0.25,11.8,9.5));
#7964=CARTESIAN_POINT('',(-0.25,11.8,8.8));
#7965=CARTESIAN_POINT('Origin',(0.,11.8,9.5));
#7966=CARTESIAN_POINT('Origin',(0.,11.8,8.2));
#7967=CARTESIAN_POINT('',(-0.2,11.8,8.2));
#7968=CARTESIAN_POINT('Origin',(0.,11.8,8.2));
#7969=CARTESIAN_POINT('Origin',(0.,11.8,7.5));
#7970=CARTESIAN_POINT('',(-1.,11.7820508075689,7.5));
#7971=CARTESIAN_POINT('',(-0.505181485540923,10.925,7.5));
#7972=CARTESIAN_POINT('',(-1.01036297108185,11.8,7.5));
#7973=CARTESIAN_POINT('',(0.505181485540923,10.925,7.5));
#7974=CARTESIAN_POINT('',(-0.505181485540923,10.925,7.5));
#7975=CARTESIAN_POINT('',(1.,11.7820508075689,7.5));
#7976=CARTESIAN_POINT('',(0.505181485540923,10.925,7.5));
#7977=CARTESIAN_POINT('',(1.,10.8,7.5));
#7978=CARTESIAN_POINT('',(1.,10.8,7.5));
#7979=CARTESIAN_POINT('',(-1.,10.8,7.5));
#7980=CARTESIAN_POINT('',(-1.,10.8,7.5));
#7981=CARTESIAN_POINT('',(-1.,12.8,7.5));
#7982=CARTESIAN_POINT('Origin',(1.,12.8,7.5));
#7983=CARTESIAN_POINT('',(1.,12.8,7.5));
#7984=CARTESIAN_POINT('',(-1.,12.8,7.5));
#7985=CARTESIAN_POINT('',(1.,12.8,7.5));
#7986=CARTESIAN_POINT('',(-1.,12.8,9.5));
#7987=CARTESIAN_POINT('',(-1.,12.8,7.5));
#7988=CARTESIAN_POINT('',(1.,12.8,9.5));
#7989=CARTESIAN_POINT('',(1.,12.8,9.5));
#7990=CARTESIAN_POINT('',(1.,12.8,7.5));
#7991=CARTESIAN_POINT('Origin',(1.,10.8,7.5));
#7992=CARTESIAN_POINT('',(1.,11.8179491924311,7.5));
#7993=CARTESIAN_POINT('',(1.,11.3,7.5));
#7994=CARTESIAN_POINT('',(1.,10.8,7.5));
#7995=CARTESIAN_POINT('',(1.,10.8,9.5));
#7996=CARTESIAN_POINT('',(1.,10.8,9.5));
#7997=CARTESIAN_POINT('',(1.,10.8,7.5));
#7998=CARTESIAN_POINT('Origin',(-1.,10.8,7.5));
#7999=CARTESIAN_POINT('',(-1.,10.8,9.5));
#8000=CARTESIAN_POINT('',(-1.,10.8,9.5));
#8001=CARTESIAN_POINT('',(-1.,10.8,7.5));
#8002=CARTESIAN_POINT('Origin',(-1.,12.8,7.5));
#8003=CARTESIAN_POINT('',(-1.,11.8179491924311,7.5));
#8004=CARTESIAN_POINT('',(-1.,12.8,7.5));
#8005=CARTESIAN_POINT('',(-1.,12.3,7.5));
#8006=CARTESIAN_POINT('',(-1.,12.8,9.5));
#8007=CARTESIAN_POINT('Origin',(0.,11.8,9.5));
#8008=CARTESIAN_POINT('Origin',(0.,11.8,7.5));
#8009=CARTESIAN_POINT('',(-0.505181485540922,12.675,7.5));
#8010=CARTESIAN_POINT('',(-0.505181485540922,12.675,7.5));
#8011=CARTESIAN_POINT('',(0.505181485540923,12.675,7.5));
#8012=CARTESIAN_POINT('',(1.01036297108185,11.8,7.5));
#8013=CARTESIAN_POINT('',(0.505181485540923,12.675,7.5));
#8014=CARTESIAN_POINT('Origin',(0.,11.8,7.5));
#8015=CARTESIAN_POINT('',(1.01036297108185,11.8,7.5));
#8016=CARTESIAN_POINT('',(0.505181485540923,10.925,7.5));
#8017=CARTESIAN_POINT('',(1.01036297108185,11.8,7.5));
#8018=CARTESIAN_POINT('Origin',(0.,11.8,7.));
#8019=CARTESIAN_POINT('',(0.505181485540923,10.925,7.));
#8020=CARTESIAN_POINT('',(1.01036297108185,11.8,7.));
#8021=CARTESIAN_POINT('',(0.505181485540923,10.925,7.));
#8022=CARTESIAN_POINT('',(-0.505181485540923,10.925,7.));
#8023=CARTESIAN_POINT('',(-0.505181485540923,10.925,7.));
#8024=CARTESIAN_POINT('',(-1.01036297108185,11.8,7.));
#8025=CARTESIAN_POINT('',(-1.01036297108185,11.8,7.));
#8026=CARTESIAN_POINT('',(-0.505181485540922,12.675,7.));
#8027=CARTESIAN_POINT('',(-0.505181485540922,12.675,7.));
#8028=CARTESIAN_POINT('',(0.505181485540923,12.675,7.));
#8029=CARTESIAN_POINT('',(0.505181485540923,12.675,7.));
#8030=CARTESIAN_POINT('',(1.01036297108185,11.8,7.));
#8031=CARTESIAN_POINT('',(-0.685,11.8,7.));
#8032=CARTESIAN_POINT('Origin',(0.,11.8,7.));
#8033=CARTESIAN_POINT('Origin',(-0.505181485540923,10.925,7.));
#8034=CARTESIAN_POINT('',(0.505181485540923,10.925,7.));
#8035=CARTESIAN_POINT('',(-0.505181485540923,10.925,7.));
#8036=CARTESIAN_POINT('Origin',(-1.01036297108185,11.8,7.));
#8037=CARTESIAN_POINT('',(-1.01036297108185,11.8,7.5));
#8038=CARTESIAN_POINT('',(-1.01036297108185,11.8,7.5));
#8039=CARTESIAN_POINT('',(-1.01036297108185,11.8,7.));
#8040=CARTESIAN_POINT('Origin',(-0.505181485540922,12.675,7.));
#8041=CARTESIAN_POINT('',(-0.505181485540922,12.675,7.5));
#8042=CARTESIAN_POINT('',(-0.505181485540922,12.675,7.));
#8043=CARTESIAN_POINT('Origin',(0.505181485540923,12.675,7.));
#8044=CARTESIAN_POINT('',(0.505181485540923,12.675,7.));
#8045=CARTESIAN_POINT('Origin',(1.01036297108185,11.8,7.));
#8046=CARTESIAN_POINT('',(1.01036297108185,11.8,7.));
#8047=CARTESIAN_POINT('Origin',(0.505181485540923,10.925,7.));
#8048=CARTESIAN_POINT('Origin',(0.,11.8,7.5));
#8049=CARTESIAN_POINT('Origin',(0.,11.8,5.8));
#8050=CARTESIAN_POINT('',(-0.2,11.8,5.8));
#8051=CARTESIAN_POINT('',(-0.2,11.8,5.8));
#8052=CARTESIAN_POINT('Origin',(0.,11.8,5.8));
#8053=CARTESIAN_POINT('Origin',(0.,11.8,5.8));
#8054=CARTESIAN_POINT('',(-0.685,11.8,5.8));
#8055=CARTESIAN_POINT('',(-0.685,11.8,5.8));
#8056=CARTESIAN_POINT('Origin',(0.,11.8,5.8));
#8057=CARTESIAN_POINT('Origin',(0.,11.8,5.8));
#9043=UNCERTAINTY_MEASURE_WITH_UNIT(LENGTH_MEASURE(0.001),#9103,
'DISTANCE_ACCURACY_VALUE',
'Maximum model space distance between geometric entities at asserted c
onnectivities');
#9069=UNCERTAINTY_MEASURE_WITH_UNIT(LENGTH_MEASURE(0.001),#9103,
'DISTANCE_ACCURACY_VALUE',
'Maximum model space distance between geometric entities at asserted c
onnectivities');
#9076=(
GEOMETRIC_REPRESENTATION_CONTEXT(3)
GLOBAL_UNCERTAINTY_ASSIGNED_CONTEXT((#9043))
GLOBAL_UNIT_ASSIGNED_CONTEXT((#9103,#9105,#9106))
REPRESENTATION_CONTEXT('','3D')
);
#9102=(
GEOMETRIC_REPRESENTATION_CONTEXT(3)
GLOBAL_UNCERTAINTY_ASSIGNED_CONTEXT((#9069))
GLOBAL_UNIT_ASSIGNED_CONTEXT((#9103,#9105,#9106))
REPRESENTATION_CONTEXT('','3D')
);
#9103=(
LENGTH_UNIT()
NAMED_UNIT(*)
SI_UNIT(.CENTI.,.METRE.)
);
#9105=(
NAMED_UNIT(*)
PLANE_ANGLE_UNIT()
SI_UNIT($,.RADIAN.)
);
#9106=(
NAMED_UNIT(*)
SI_UNIT($,.STERADIAN.)
SOLID_ANGLE_UNIT()
);
#9113=SHAPE_DEFINITION_REPRESENTATION(#9145,#9233);
#9145=PRODUCT_DEFINITION_SHAPE('',$,#9266);
#9233=SHAPE_REPRESENTATION('',(#5458),#9076);
#9259=PRODUCT_DEFINITION_CONTEXT('part definition',#9357,'design');
#9266=PRODUCT_DEFINITION('Needle flow-control fitting (1)',
'Needle flow-control fitting (1)',#9298,#9259);
#9298=PRODUCT_DEFINITION_FORMATION('',$,#9365);
#9357=APPLICATION_CONTEXT(
'Core Data for Automotive Mechanical Design Process');
#9358=PRODUCT_CONTEXT('part definition',#9357,'mechanical');
#9365=PRODUCT('Needle flow-control fitting (1)',
'Needle flow-control fitting (1)','Needle flow-control fitting (1)',(#9358));
#9447=COLOUR_RGB('Sky Blue',0.24,0.69,0.87);
#9448=FILL_AREA_STYLE_COLOUR('',#9447);
#9449=FILL_AREA_STYLE('',(#9448));
#9450=SURFACE_STYLE_FILL_AREA(#9449);
#9451=SURFACE_SIDE_STYLE('',(#9450));
#9452=SURFACE_STYLE_USAGE(.BOTH.,#9451);
#9453=PRESENTATION_STYLE_ASSIGNMENT((#9452));
ENDSEC;
END-ISO-10303-21;
